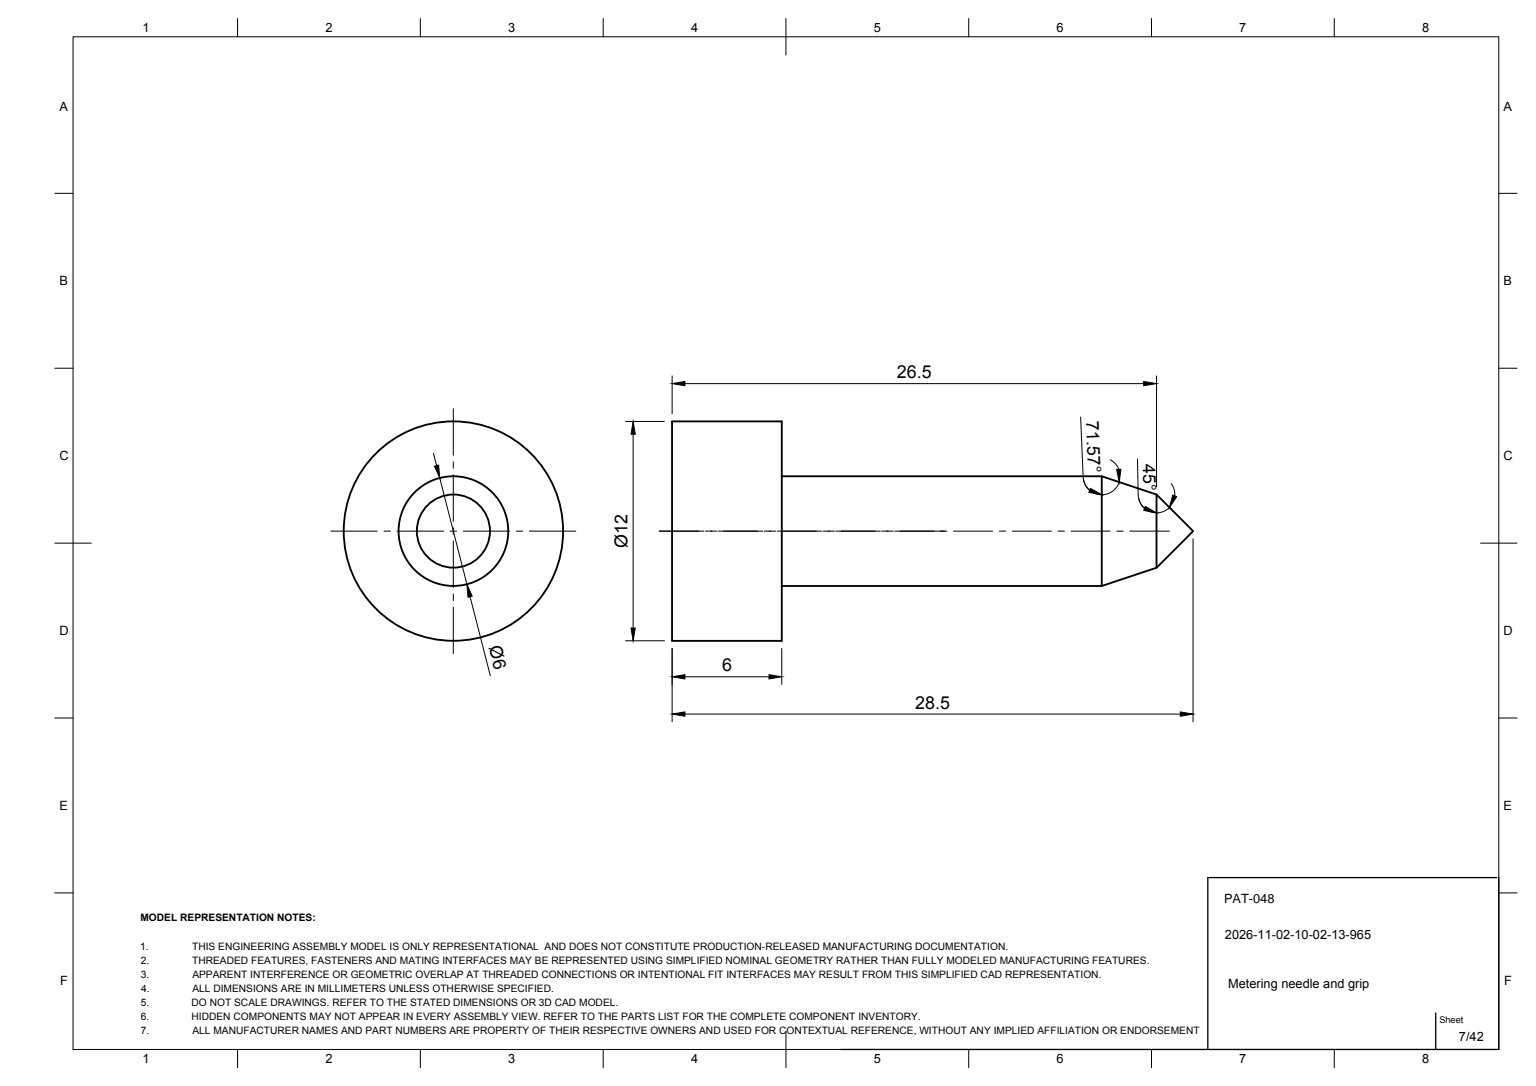
ISO-10303-21;
HEADER;
/* Generated by software containing ST-Developer
 * from STEP Tools, Inc. (www.steptools.com) 
 */

FILE_DESCRIPTION(
/* description */ ('Guided pneumatic stop gate'),
/* implementation_level */ '2;1');

FILE_NAME(
/* name */ 'Metering needle and grip.step',
/* time_stamp */ '2026-10-27T21:43:45-07:00',
/* author */ (''),
/* organization */ (''),
/* preprocessor_version */ 'ST-DEVELOPER v20.2',
/* originating_system */ 'Autodesk Translation Framework v15.17.0.0',
/* authorisation */ '');

FILE_SCHEMA (('AUTOMOTIVE_DESIGN { 1 0 10303 214 3 1 1 }'));
ENDSEC;

DATA;
#10=MECHANICAL_DESIGN_GEOMETRIC_PRESENTATION_REPRESENTATION('',(#537),#14392);
#423=CONICAL_SURFACE('',#8501,0.1,0.78539816339745);
#424=CONICAL_SURFACE('',#8503,0.25,0.321750554396641);
#453=SHAPE_REPRESENTATION_RELATIONSHIP('SRR','None',#14587,#495);
#495=ADVANCED_BREP_SHAPE_REPRESENTATION('',(#579),#14349);
#537=STYLED_ITEM('',(#14898),#579);
#579=MANIFOLD_SOLID_BREP('Body1',#7877);
#639=FACE_BOUND('',#1682,.T.);
#878=PLANE('',#8507);
#879=PLANE('',#8511);
#1179=FACE_OUTER_BOUND('',#1678,.T.);
#1180=FACE_OUTER_BOUND('',#1679,.T.);
#1181=FACE_OUTER_BOUND('',#1680,.T.);
#1182=FACE_OUTER_BOUND('',#1681,.T.);
#1183=FACE_OUTER_BOUND('',#1683,.T.);
#1184=FACE_OUTER_BOUND('',#1684,.T.);
#1678=EDGE_LOOP('',(#5574,#5575,#5576));
#1679=EDGE_LOOP('',(#5577,#5578,#5579,#5580));
#1680=EDGE_LOOP('',(#5581,#5582,#5583,#5584));
#1681=EDGE_LOOP('',(#5585));
#1682=EDGE_LOOP('',(#5586));
#1683=EDGE_LOOP('',(#5587,#5588,#5589,#5590));
#1684=EDGE_LOOP('',(#5591));
#2356=LINE('',#12199,#2901);
#2357=LINE('',#12203,#2902);
#2358=LINE('',#12207,#2903);
#2359=LINE('',#12214,#2904);
#2901=VECTOR('',#9697,0.1);
#2902=VECTOR('',#9702,0.25);
#2903=VECTOR('',#9707,0.3);
#2904=VECTOR('',#9716,0.6);
#3412=CIRCLE('',#8502,0.2);
#3413=CIRCLE('',#8504,0.3);
#3414=CIRCLE('',#8506,0.3);
#3415=CIRCLE('',#8508,0.6);
#3416=CIRCLE('',#8510,0.6);
#3817=VERTEX_POINT('',#12196);
#3818=VERTEX_POINT('',#12198);
#3819=VERTEX_POINT('',#12201);
#3820=VERTEX_POINT('',#12205);
#3821=VERTEX_POINT('',#12209);
#3822=VERTEX_POINT('',#12212);
#4485=EDGE_CURVE('',#3817,#3817,#3412,.T.);
#4486=EDGE_CURVE('',#3817,#3818,#2356,.T.);
#4487=EDGE_CURVE('',#3819,#3819,#3413,.T.);
#4488=EDGE_CURVE('',#3819,#3817,#2357,.T.);
#4489=EDGE_CURVE('',#3820,#3820,#3414,.T.);
#4490=EDGE_CURVE('',#3820,#3819,#2358,.T.);
#4491=EDGE_CURVE('',#3821,#3821,#3415,.T.);
#4492=EDGE_CURVE('',#3822,#3822,#3416,.T.);
#4493=EDGE_CURVE('',#3822,#3821,#2359,.T.);
#5574=ORIENTED_EDGE('',*,*,#4485,.F.);
#5575=ORIENTED_EDGE('',*,*,#4486,.T.);
#5576=ORIENTED_EDGE('',*,*,#4486,.F.);
#5577=ORIENTED_EDGE('',*,*,#4487,.F.);
#5578=ORIENTED_EDGE('',*,*,#4488,.T.);
#5579=ORIENTED_EDGE('',*,*,#4485,.T.);
#5580=ORIENTED_EDGE('',*,*,#4488,.F.);
#5581=ORIENTED_EDGE('',*,*,#4489,.F.);
#5582=ORIENTED_EDGE('',*,*,#4490,.T.);
#5583=ORIENTED_EDGE('',*,*,#4487,.T.);
#5584=ORIENTED_EDGE('',*,*,#4490,.F.);
#5585=ORIENTED_EDGE('',*,*,#4491,.F.);
#5586=ORIENTED_EDGE('',*,*,#4489,.T.);
#5587=ORIENTED_EDGE('',*,*,#4492,.F.);
#5588=ORIENTED_EDGE('',*,*,#4493,.T.);
#5589=ORIENTED_EDGE('',*,*,#4491,.T.);
#5590=ORIENTED_EDGE('',*,*,#4493,.F.);
#5591=ORIENTED_EDGE('',*,*,#4492,.T.);
#7258=CYLINDRICAL_SURFACE('',#8505,0.3);
#7259=CYLINDRICAL_SURFACE('',#8509,0.6);
#7461=ADVANCED_FACE('',(#1179),#423,.T.);
#7462=ADVANCED_FACE('',(#1180),#424,.T.);
#7463=ADVANCED_FACE('',(#1181),#7258,.T.);
#7464=ADVANCED_FACE('',(#1182,#639),#878,.T.);
#7465=ADVANCED_FACE('',(#1183),#7259,.T.);
#7466=ADVANCED_FACE('',(#1184),#879,.T.);
#7877=CLOSED_SHELL('',(#7461,#7462,#7463,#7464,#7465,#7466));
#8500=AXIS2_PLACEMENT_3D('',#12194,#9691,#9692);
#8501=AXIS2_PLACEMENT_3D('',#12195,#9693,#9694);
#8502=AXIS2_PLACEMENT_3D('',#12197,#9695,#9696);
#8503=AXIS2_PLACEMENT_3D('',#12200,#9698,#9699);
#8504=AXIS2_PLACEMENT_3D('',#12202,#9700,#9701);
#8505=AXIS2_PLACEMENT_3D('',#12204,#9703,#9704);
#8506=AXIS2_PLACEMENT_3D('',#12206,#9705,#9706);
#8507=AXIS2_PLACEMENT_3D('',#12208,#9708,#9709);
#8508=AXIS2_PLACEMENT_3D('',#12210,#9710,#9711);
#8509=AXIS2_PLACEMENT_3D('',#12211,#9712,#9713);
#8510=AXIS2_PLACEMENT_3D('',#12213,#9714,#9715);
#8511=AXIS2_PLACEMENT_3D('',#12215,#9717,#9718);
#9691=DIRECTION('axis',(0.,0.,1.));
#9692=DIRECTION('refdir',(1.,0.,0.));
#9693=DIRECTION('center_axis',(0.,0.,1.));
#9694=DIRECTION('ref_axis',(1.,0.,0.));
#9695=DIRECTION('center_axis',(0.,0.,1.));
#9696=DIRECTION('ref_axis',(1.,0.,0.));
#9697=DIRECTION('',(0.707106781186549,8.65956056235495E-17,-0.707106781186546));
#9698=DIRECTION('center_axis',(0.,0.,1.));
#9699=DIRECTION('ref_axis',(1.,0.,0.));
#9700=DIRECTION('center_axis',(0.,0.,1.));
#9701=DIRECTION('ref_axis',(1.,0.,0.));
#9702=DIRECTION('',(0.316227766016837,3.87267321454038E-17,-0.948683298050514));
#9703=DIRECTION('center_axis',(0.,0.,1.));
#9704=DIRECTION('ref_axis',(1.,0.,0.));
#9705=DIRECTION('center_axis',(0.,0.,1.));
#9706=DIRECTION('ref_axis',(1.,0.,0.));
#9707=DIRECTION('',(0.,0.,-1.));
#9708=DIRECTION('center_axis',(0.,0.,-1.));
#9709=DIRECTION('ref_axis',(-1.,0.,0.));
#9710=DIRECTION('center_axis',(0.,0.,1.));
#9711=DIRECTION('ref_axis',(1.,0.,0.));
#9712=DIRECTION('center_axis',(0.,0.,1.));
#9713=DIRECTION('ref_axis',(1.,0.,0.));
#9714=DIRECTION('center_axis',(0.,0.,1.));
#9715=DIRECTION('ref_axis',(1.,0.,0.));
#9716=DIRECTION('',(0.,0.,-1.));
#9717=DIRECTION('center_axis',(0.,0.,1.));
#9718=DIRECTION('ref_axis',(1.,0.,0.));
#12194=CARTESIAN_POINT('',(0.,0.,0.));
#12195=CARTESIAN_POINT('Origin',(0.,0.8,8.15));
#12196=CARTESIAN_POINT('',(-0.2,0.8,8.25));
#12197=CARTESIAN_POINT('Origin',(0.,0.8,8.25));
#12198=CARTESIAN_POINT('',(0.,0.8,8.05));
#12199=CARTESIAN_POINT('',(-0.1,0.8,8.15));
#12200=CARTESIAN_POINT('Origin',(0.,0.8,8.4));
#12201=CARTESIAN_POINT('',(-0.3,0.8,8.55));
#12202=CARTESIAN_POINT('Origin',(0.,0.8,8.55));
#12203=CARTESIAN_POINT('',(-0.25,0.8,8.4));
#12204=CARTESIAN_POINT('Origin',(0.,0.8,9.425));
#12205=CARTESIAN_POINT('',(-0.3,0.8,10.3));
#12206=CARTESIAN_POINT('Origin',(0.,0.8,10.3));
#12207=CARTESIAN_POINT('',(-0.3,0.8,9.425));
#12208=CARTESIAN_POINT('Origin',(0.6,0.8,10.3));
#12209=CARTESIAN_POINT('',(-0.6,0.8,10.3));
#12210=CARTESIAN_POINT('Origin',(0.,0.8,10.3));
#12211=CARTESIAN_POINT('Origin',(0.,0.8,10.6));
#12212=CARTESIAN_POINT('',(-0.6,0.8,10.9));
#12213=CARTESIAN_POINT('Origin',(0.,0.8,10.9));
#12214=CARTESIAN_POINT('',(-0.6,0.8,10.6));
#12215=CARTESIAN_POINT('Origin',(0.,0.8,10.9));
#14301=UNCERTAINTY_MEASURE_WITH_UNIT(LENGTH_MEASURE(0.001),#14393,
'DISTANCE_ACCURACY_VALUE',
'Maximum model space distance between geometric entities at asserted c
onnectivities');
#14344=UNCERTAINTY_MEASURE_WITH_UNIT(LENGTH_MEASURE(0.001),#14393,
'DISTANCE_ACCURACY_VALUE',
'Maximum model space distance between geometric entities at asserted c
onnectivities');
#14349=(
GEOMETRIC_REPRESENTATION_CONTEXT(3)
GLOBAL_UNCERTAINTY_ASSIGNED_CONTEXT((#14301))
GLOBAL_UNIT_ASSIGNED_CONTEXT((#14393,#14395,#14396))
REPRESENTATION_CONTEXT('','3D')
);
#14392=(
GEOMETRIC_REPRESENTATION_CONTEXT(3)
GLOBAL_UNCERTAINTY_ASSIGNED_CONTEXT((#14344))
GLOBAL_UNIT_ASSIGNED_CONTEXT((#14393,#14395,#14396))
REPRESENTATION_CONTEXT('','3D')
);
#14393=(
LENGTH_UNIT()
NAMED_UNIT(*)
SI_UNIT(.CENTI.,.METRE.)
);
#14395=(
NAMED_UNIT(*)
PLANE_ANGLE_UNIT()
SI_UNIT($,.RADIAN.)
);
#14396=(
NAMED_UNIT(*)
SI_UNIT($,.STERADIAN.)
SOLID_ANGLE_UNIT()
);
#14401=SHAPE_DEFINITION_REPRESENTATION(#14448,#14587);
#14448=PRODUCT_DEFINITION_SHAPE('',$,#14635);
#14587=SHAPE_REPRESENTATION('',(#8500),#14349);
#14630=PRODUCT_DEFINITION_CONTEXT('part definition',#14773,'design');
#14635=PRODUCT_DEFINITION('Metering needle and grip',
'Metering needle and grip',#14682,#14630);
#14682=PRODUCT_DEFINITION_FORMATION('',$,#14779);
#14773=APPLICATION_CONTEXT(
'Core Data for Automotive Mechanical Design Process');
#14774=PRODUCT_CONTEXT('part definition',#14773,'mechanical');
#14779=PRODUCT('Metering needle and grip','Metering needle and grip',
'Metering needle and grip',(#14774));
#14892=COLOUR_RGB('Black',0.12,0.14,0.17);
#14893=FILL_AREA_STYLE_COLOUR('',#14892);
#14894=FILL_AREA_STYLE('',(#14893));
#14895=SURFACE_STYLE_FILL_AREA(#14894);
#14896=SURFACE_SIDE_STYLE('',(#14895));
#14897=SURFACE_STYLE_USAGE(.BOTH.,#14896);
#14898=PRESENTATION_STYLE_ASSIGNMENT((#14897));
ENDSEC;
END-ISO-10303-21;
